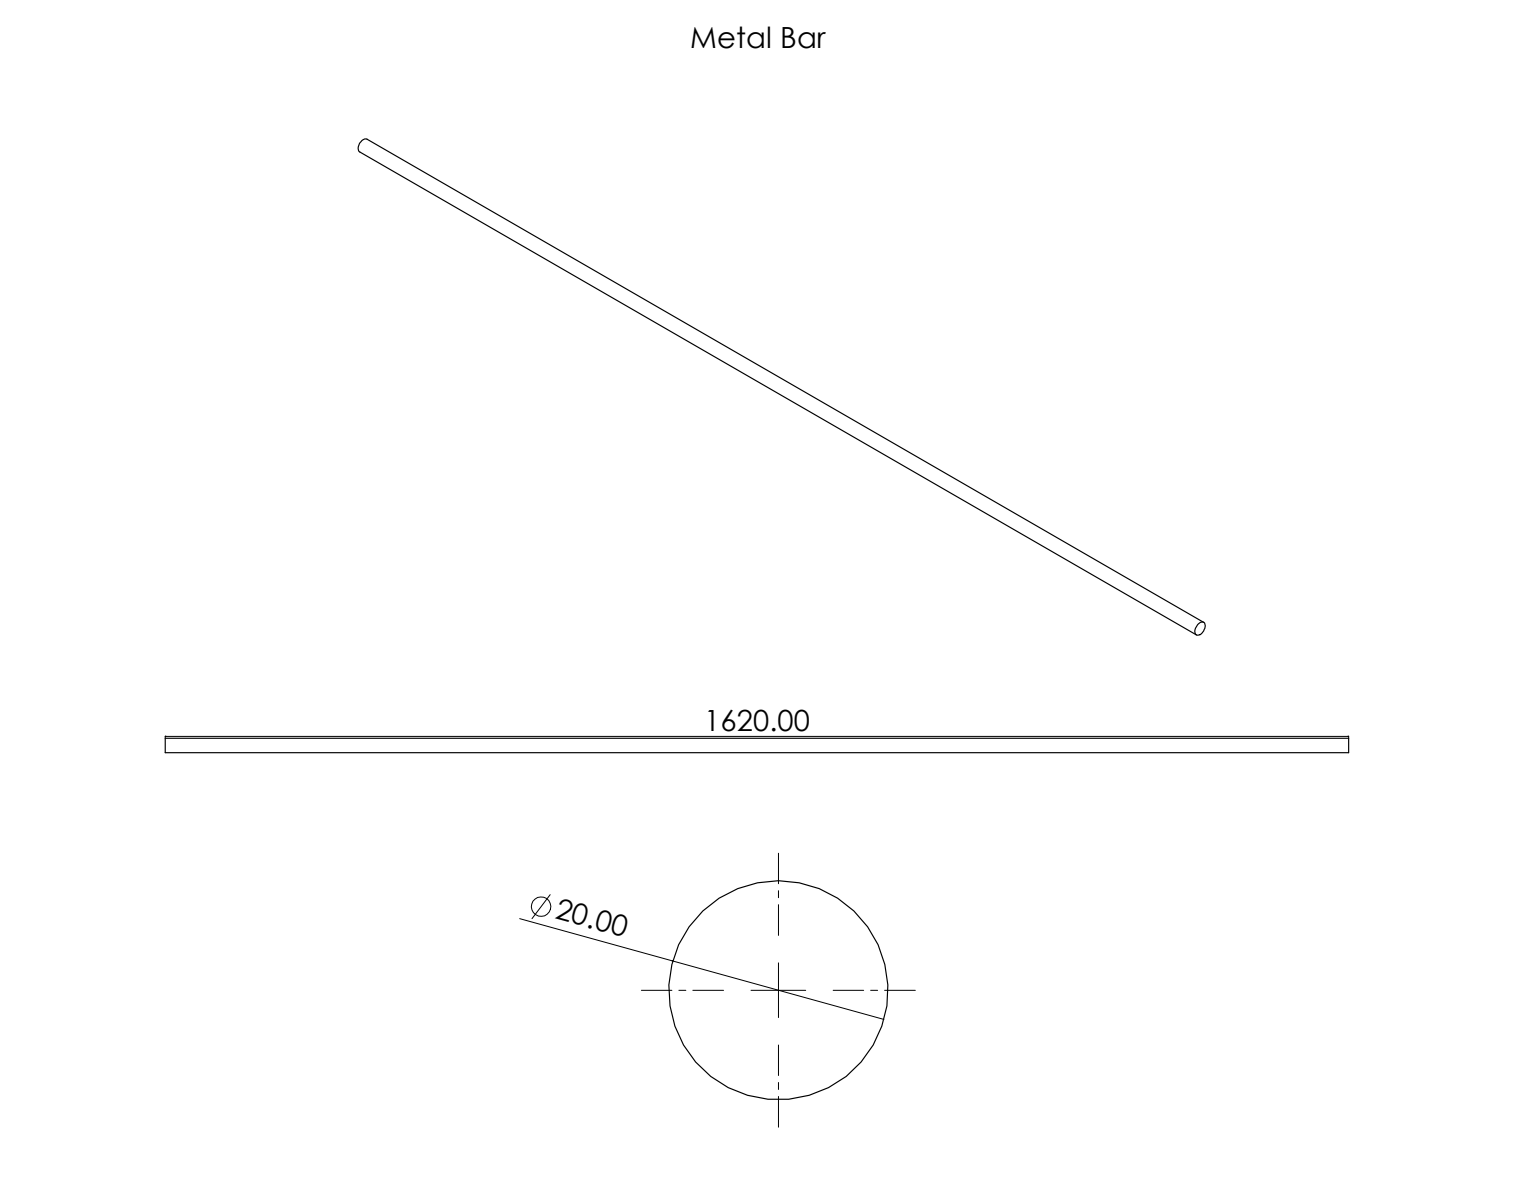
ISO-10303-21;
HEADER;
FILE_DESCRIPTION (('STEP AP214'),
    '1' );
FILE_NAME ('Metal Bar.step',
    '2026-10-21T17:07:05',
    ( '' ),
    ( '' ),
    'SwSTEP 2.0',
    'SolidWorks 2025',
    '' );
FILE_SCHEMA (( 'AUTOMOTIVE_DESIGN' ));
ENDSEC;

DATA;
#79=PRODUCT ( 'Metal Bar', 'Metal Bar', '', ( #35741 ) ) ;
#543=LINE ( 'NONE', #39589, #26981 ) ;
#549=ORIENTED_EDGE ( 'NONE', *, *, #40552, .F. ) ;
#700=CARTESIAN_POINT ( 'NONE',  ( 809.9999999999993179, -512.9681489794448908, -339.9999999999999432 ) ) ;
#1022=UNCERTAINTY_MEASURE_WITH_UNIT (LENGTH_MEASURE( 1.000000000000000082E-05 ), #11175, 'distance_accuracy_value', 'NONE');
#1024=DIRECTION ( 'NONE',  ( -1.000000000000000000, -0.000000000000000000, 0.000000000000000000 ) ) ;
#2121=CARTESIAN_POINT ( 'NONE',  ( 809.9999999999993179, -512.9681489794448908, -329.9999999999999432 ) ) ;
#2779=CYLINDRICAL_SURFACE ( 'NONE', #28718, 10.00000000000000888 ) ;
#3333=DIRECTION ( 'NONE',  ( 1.000000000000000000, 0.000000000000000000, -0.000000000000000000 ) ) ;
#3764=SHAPE_REPRESENTATION_RELATIONSHIP ( 'NONE' , 'NONE' ,  #15645, #8939 ) ;
#3940=EDGE_LOOP ( 'NONE', ( #39481, #22505 ) ) ;
#4013=( NAMED_UNIT ( * ) PLANE_ANGLE_UNIT ( ) SI_UNIT ( $, .RADIAN. ) );
#4259=( NAMED_UNIT ( * ) SI_UNIT ( $, .STERADIAN. ) SOLID_ANGLE_UNIT ( ) );
#5266=VERTEX_POINT ( 'NONE', #2121 ) ;
#6075=DIRECTION ( 'NONE',  ( 1.000000000000000000, 0.000000000000000000, 0.000000000000000000 ) ) ;
#7190=EDGE_LOOP ( 'NONE', ( #42020, #36578, #13036, #37313 ) ) ;
#7222=APPLICATION_CONTEXT ( 'automotive_design' ) ;
#7432=CARTESIAN_POINT ( 'NONE',  ( -809.9999999999993179, -512.9681489794448908, -350.0000000000000000 ) ) ;
#7841=VERTEX_POINT ( 'NONE', #7432 ) ;
#8092=AXIS2_PLACEMENT_3D ( 'NONE', #39555, #40221, #21980 ) ;
#8163=DIRECTION ( 'NONE',  ( 1.000000000000000000, -0.000000000000000000, -0.000000000000000000 ) ) ;
#8611=ORIENTED_EDGE ( 'NONE', *, *, #36003, .F. ) ;
#8815=CARTESIAN_POINT ( 'NONE',  ( -809.9999999999993179, -512.9681489794448908, -329.9999999999999432 ) ) ;
#8939=ADVANCED_BREP_SHAPE_REPRESENTATION ( '', ( #16696, #26858 ), #23892 ) ;
#9050=MECHANICAL_DESIGN_GEOMETRIC_PRESENTATION_REPRESENTATION('',(#9778),#44465);
#9778=STYLED_ITEM('',(#45751),#16696);
#9818=CARTESIAN_POINT ( 'NONE',  ( -809.9999999999993179, -512.9681489794448908, -339.9999999999999432 ) ) ;
#10159=CARTESIAN_POINT ( 'NONE',  ( -809.9999999999993179, -512.9681489794448908, -339.9999999999999432 ) ) ;
#10459=EDGE_CURVE ( 'NONE', #35164, #5266, #543, .T. ) ;
#10816=SHAPE_DEFINITION_REPRESENTATION ( #35485, #15645 ) ;
#11175=( LENGTH_UNIT ( ) NAMED_UNIT ( * ) SI_UNIT ( .MILLI., .METRE. ) );
#13036=ORIENTED_EDGE ( 'NONE', *, *, #16452, .F. ) ;
#14406=FACE_OUTER_BOUND ( 'NONE', #7190, .T. ) ;
#14902=FACE_OUTER_BOUND ( 'NONE', #25277, .T. ) ;
#15363=EDGE_LOOP ( 'NONE', ( #22382, #549, #26810, #8611 ) ) ;
#15645=SHAPE_REPRESENTATION ( 'Metal Bar', ( #26858 ), #23892 ) ;
#15739=AXIS2_PLACEMENT_3D ( 'NONE', #35347, #18285, #17586 ) ;
#15817=CARTESIAN_POINT ( 'NONE',  ( 809.9999999999993179, -512.9681489794448908, -350.0000000000000000 ) ) ;
#16452=EDGE_CURVE ( 'NONE', #42952, #5266, #26721, .T. ) ;
#16497=CIRCLE ( 'NONE', #15739, 10.00000000000000888 ) ;
#16696=MANIFOLD_SOLID_BREP ( 'Boss-Extrude23', #32822 ) ;
#16761=PLANE ( 'NONE',  #27655 ) ;
#17586=DIRECTION ( 'NONE',  ( 0.000000000000000000, 0.000000000000000000, 1.000000000000000000 ) ) ;
#17962=CARTESIAN_POINT ( 'NONE',  ( -809.9999999999993179, -512.9681489794448908, -350.0000000000000000 ) ) ;
#18285=DIRECTION ( 'NONE',  ( -1.000000000000000000, 0.000000000000000000, 0.000000000000000000 ) ) ;
#18339=DIRECTION ( 'NONE',  ( 1.000000000000000000, -0.000000000000000000, -0.000000000000000000 ) ) ;
#18424=LINE ( 'NONE', #17962, #43022 ) ;
#21088=( NAMED_UNIT ( * ) SI_UNIT ( $, .STERADIAN. ) SOLID_ANGLE_UNIT ( ) );
#21922=ADVANCED_FACE ( 'NONE', ( #41701 ), #16761, .T. ) ;
#21980=DIRECTION ( 'NONE',  ( 0.000000000000000000, 0.000000000000000000, 1.000000000000000000 ) ) ;
#22382=ORIENTED_EDGE ( 'NONE', *, *, #10459, .F. ) ;
#22505=ORIENTED_EDGE ( 'NONE', *, *, #37682, .T. ) ;
#22716=UNCERTAINTY_MEASURE_WITH_UNIT (LENGTH_MEASURE( 1.000000000000000082E-05 ), #35391, 'distance_accuracy_value', 'NONE');
#23153=CARTESIAN_POINT ( 'NONE',  ( 0.000000000000000000, 0.000000000000000000, 0.000000000000000000 ) ) ;
#23707=APPLICATION_CONTEXT ( 'automotive_design' ) ;
#23840=( NAMED_UNIT ( * ) PLANE_ANGLE_UNIT ( ) SI_UNIT ( $, .RADIAN. ) );
#23892=( GEOMETRIC_REPRESENTATION_CONTEXT ( 3 ) GLOBAL_UNCERTAINTY_ASSIGNED_CONTEXT ( ( #22716 ) ) GLOBAL_UNIT_ASSIGNED_CONTEXT ( ( #35391, #23840, #21088 ) ) REPRESENTATION_CONTEXT ( 'NONE', 'WORKASPACE' ) );
#24923=DIRECTION ( 'NONE',  ( 1.000000000000000000, -0.000000000000000000, -0.000000000000000000 ) ) ;
#25017=CARTESIAN_POINT ( 'NONE',  ( -809.9999999999993179, -512.9681489794448908, -339.9999999999999432 ) ) ;
#25277=EDGE_LOOP ( 'NONE', ( #27427, #33103 ) ) ;
#25299=PRODUCT_DEFINITION_FORMATION_WITH_SPECIFIED_SOURCE ( 'ANY', '', #79, .NOT_KNOWN. ) ;
#25395=DIRECTION ( 'NONE',  ( 1.000000000000000000, 0.000000000000000000, -0.000000000000000000 ) ) ;
#25705=DIRECTION ( 'NONE',  ( 0.000000000000000000, 0.000000000000000000, -1.000000000000000000 ) ) ;
#26721=CIRCLE ( 'NONE', #28950, 10.00000000000000888 ) ;
#26810=ORIENTED_EDGE ( 'NONE', *, *, #33110, .T. ) ;
#26858=AXIS2_PLACEMENT_3D ( 'NONE', #23153, #34241, #6075 ) ;
#26981=VECTOR ( 'NONE', #18339, 1000.000000000000000 ) ;
#27427=ORIENTED_EDGE ( 'NONE', *, *, #16452, .T. ) ;
#27655=AXIS2_PLACEMENT_3D ( 'NONE', #9818, #34978, #34751 ) ;
#28385=DIRECTION ( 'NONE',  ( 0.000000000000000000, 0.000000000000000000, -1.000000000000000000 ) ) ;
#28718=AXIS2_PLACEMENT_3D ( 'NONE', #10159, #24923, #28385 ) ;
#28950=AXIS2_PLACEMENT_3D ( 'NONE', #45141, #3333, #38215 ) ;
#29216=CARTESIAN_POINT ( 'NONE',  ( 809.9999999999993179, -512.9681489794448908, -339.9999999999999432 ) ) ;
#29437=DIRECTION ( 'NONE',  ( 0.000000000000000000, 0.000000000000000000, 1.000000000000000000 ) ) ;
#30917=CIRCLE ( 'NONE', #8092, 10.00000000000000888 ) ;
#31863=DIRECTION ( 'NONE',  ( 0.000000000000000000, 0.000000000000000000, 1.000000000000000000 ) ) ;
#32031=DIRECTION ( 'NONE',  ( 1.000000000000000000, -0.000000000000000000, -0.000000000000000000 ) ) ;
#32822=CLOSED_SHELL ( 'NONE', ( #39335, #38204, #21922, #33943 ) ) ;
#33103=ORIENTED_EDGE ( 'NONE', *, *, #36003, .T. ) ;
#33110=EDGE_CURVE ( 'NONE', #7841, #42952, #18424, .T. ) ;
#33943=ADVANCED_FACE ( 'NONE', ( #14902 ), #35910, .F. ) ;
#34241=DIRECTION ( 'NONE',  ( 0.000000000000000000, 0.000000000000000000, 1.000000000000000000 ) ) ;
#34751=DIRECTION ( 'NONE',  ( 0.000000000000000000, 0.000000000000000000, 1.000000000000000000 ) ) ;
#34978=DIRECTION ( 'NONE',  ( -1.000000000000000000, 0.000000000000000000, 0.000000000000000000 ) ) ;
#35164=VERTEX_POINT ( 'NONE', #8815 ) ;
#35347=CARTESIAN_POINT ( 'NONE',  ( -809.9999999999993179, -512.9681489794448908, -339.9999999999999432 ) ) ;
#35391=( LENGTH_UNIT ( ) NAMED_UNIT ( * ) SI_UNIT ( .MILLI., .METRE. ) );
#35485=PRODUCT_DEFINITION_SHAPE ( 'NONE', 'NONE',  #36333 ) ;
#35741=PRODUCT_CONTEXT ( 'NONE', #23707, 'mechanical' ) ;
#35910=PLANE ( 'NONE',  #40398 ) ;
#36003=EDGE_CURVE ( 'NONE', #5266, #42952, #39722, .T. ) ;
#36333=PRODUCT_DEFINITION ( 'UNKNOWN', '', #25299, #38575 ) ;
#36578=ORIENTED_EDGE ( 'NONE', *, *, #10459, .T. ) ;
#37313=ORIENTED_EDGE ( 'NONE', *, *, #33110, .F. ) ;
#37682=EDGE_CURVE ( 'NONE', #35164, #7841, #30917, .T. ) ;
#38204=ADVANCED_FACE ( 'NONE', ( #45266 ), #2779, .T. ) ;
#38215=DIRECTION ( 'NONE',  ( 0.000000000000000000, 0.000000000000000000, 1.000000000000000000 ) ) ;
#38575=PRODUCT_DEFINITION_CONTEXT ( 'detailed design', #7222, 'design' ) ;
#38903=CYLINDRICAL_SURFACE ( 'NONE', #44779, 10.00000000000000888 ) ;
#39335=ADVANCED_FACE ( 'NONE', ( #14406 ), #38903, .T. ) ;
#39481=ORIENTED_EDGE ( 'NONE', *, *, #40552, .T. ) ;
#39555=CARTESIAN_POINT ( 'NONE',  ( -809.9999999999993179, -512.9681489794448908, -339.9999999999999432 ) ) ;
#39589=CARTESIAN_POINT ( 'NONE',  ( -809.9999999999993179, -512.9681489794448908, -329.9999999999999432 ) ) ;
#39722=CIRCLE ( 'NONE', #44125, 10.00000000000000888 ) ;
#40221=DIRECTION ( 'NONE',  ( -1.000000000000000000, 0.000000000000000000, 0.000000000000000000 ) ) ;
#40398=AXIS2_PLACEMENT_3D ( 'NONE', #29216, #1024, #29437 ) ;
#40552=EDGE_CURVE ( 'NONE', #7841, #35164, #16497, .T. ) ;
#41701=FACE_OUTER_BOUND ( 'NONE', #3940, .T. ) ;
#42020=ORIENTED_EDGE ( 'NONE', *, *, #37682, .F. ) ;
#42952=VERTEX_POINT ( 'NONE', #15817 ) ;
#43022=VECTOR ( 'NONE', #32031, 1000.000000000000000 ) ;
#44125=AXIS2_PLACEMENT_3D ( 'NONE', #700, #25395, #31863 ) ;
#44465=( GEOMETRIC_REPRESENTATION_CONTEXT ( 3 ) GLOBAL_UNCERTAINTY_ASSIGNED_CONTEXT ( ( #1022 ) ) GLOBAL_UNIT_ASSIGNED_CONTEXT ( ( #11175, #4013, #4259 ) ) REPRESENTATION_CONTEXT ( 'NONE', 'WORKASPACE' ) );
#44779=AXIS2_PLACEMENT_3D ( 'NONE', #25017, #8163, #25705 ) ;
#45141=CARTESIAN_POINT ( 'NONE',  ( 809.9999999999993179, -512.9681489794448908, -339.9999999999999432 ) ) ;
#45266=FACE_OUTER_BOUND ( 'NONE', #15363, .T. ) ;
#45745=COLOUR_RGB('Light Blue',0.38,0.62,0.78);
#45746=FILL_AREA_STYLE_COLOUR('',#45745);
#45747=FILL_AREA_STYLE('',(#45746));
#45748=SURFACE_STYLE_FILL_AREA(#45747);
#45749=SURFACE_SIDE_STYLE('',(#45748));
#45750=SURFACE_STYLE_USAGE(.BOTH.,#45749);
#45751=PRESENTATION_STYLE_ASSIGNMENT((#45750));
ENDSEC;
END-ISO-10303-21;
